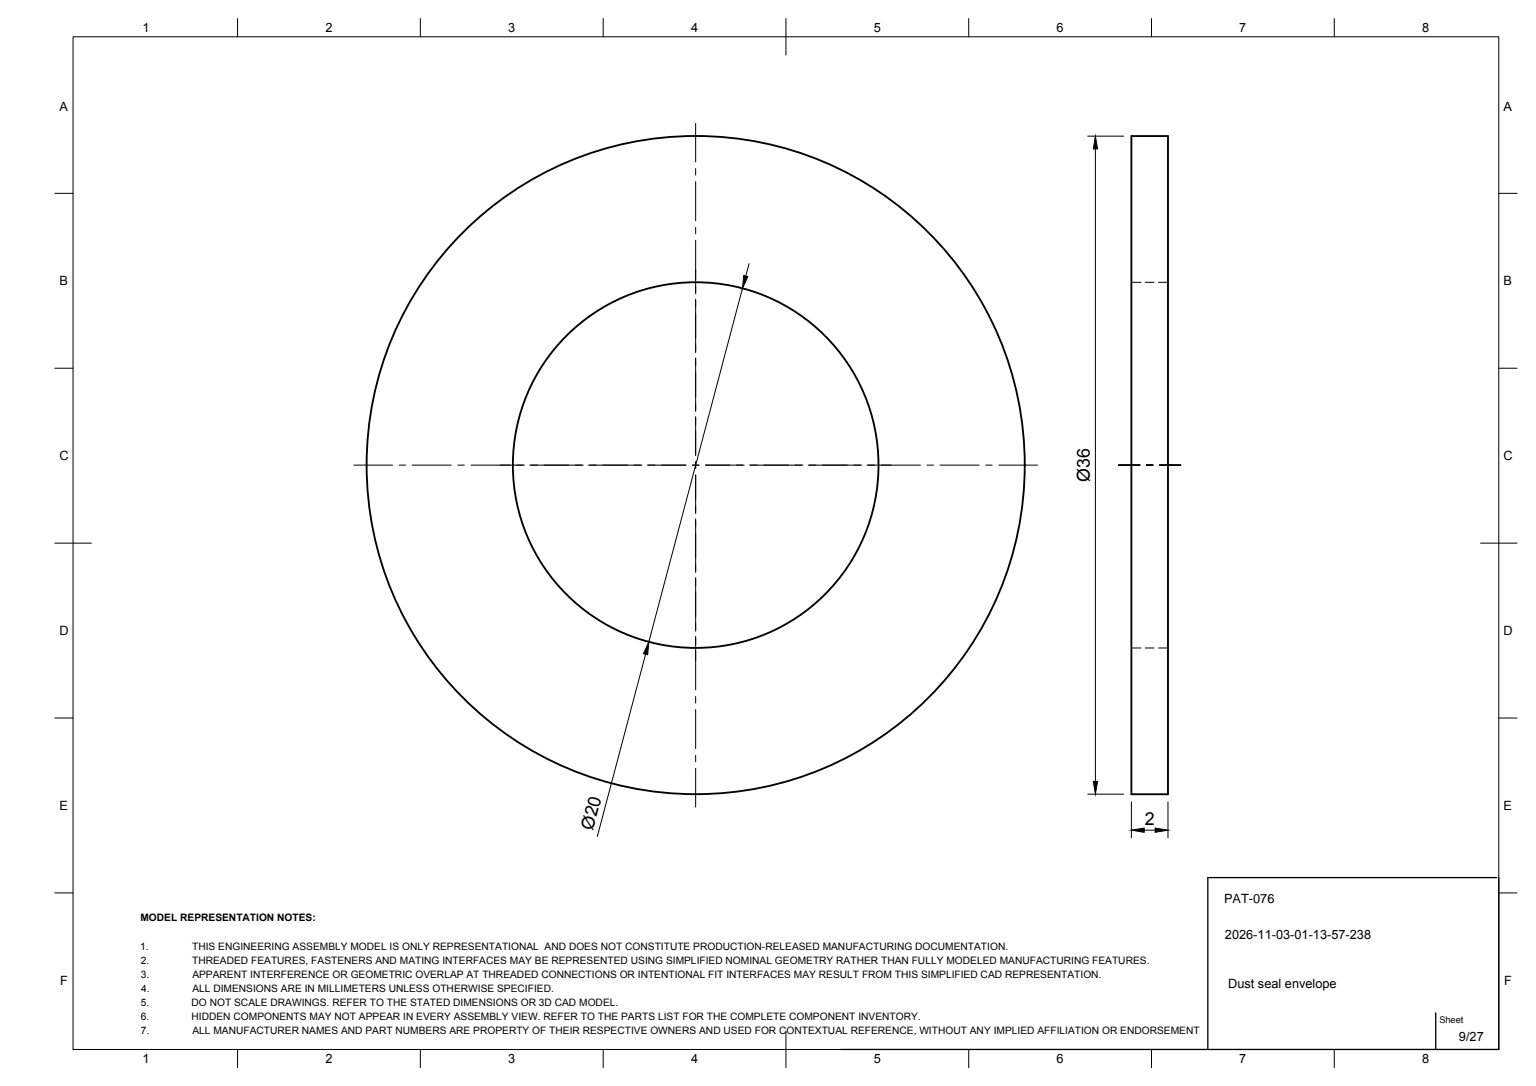
ISO-10303-21;
HEADER;
/* Generated by software containing ST-Developer
 * from STEP Tools, Inc. (www.steptools.com) 
 */

FILE_DESCRIPTION(
/* description */ ('Overhung pulley bearing cartridge'),
/* implementation_level */ '2;1');

FILE_NAME(
/* name */ 'Dust seal envelope.step',
/* time_stamp */ '2026-10-28T03:22:33-07:00',
/* author */ (''),
/* organization */ (''),
/* preprocessor_version */ 'ST-DEVELOPER v20.2',
/* originating_system */ 'Autodesk Translation Framework v15.17.0.0',
/* authorisation */ '');

FILE_SCHEMA (('AUTOMOTIVE_DESIGN { 1 0 10303 214 3 1 1 }'));
ENDSEC;

DATA;
#10=MECHANICAL_DESIGN_GEOMETRIC_PRESENTATION_REPRESENTATION('',(#287),#10963);
#243=SHAPE_REPRESENTATION_RELATIONSHIP('SRR','None',#11063,#265);
#265=ADVANCED_BREP_SHAPE_REPRESENTATION('',(#317),#10943);
#287=STYLED_ITEM('',(#11260),#317);
#317=MANIFOLD_SOLID_BREP('Body1',#5654);
#383=FACE_BOUND('',#1019,.T.);
#384=FACE_BOUND('',#1021,.T.);
#474=PLANE('',#6070);
#475=PLANE('',#6071);
#645=FACE_OUTER_BOUND('',#1016,.T.);
#646=FACE_OUTER_BOUND('',#1017,.T.);
#647=FACE_OUTER_BOUND('',#1018,.T.);
#648=FACE_OUTER_BOUND('',#1020,.T.);
#1016=EDGE_LOOP('',(#3933,#3934,#3935,#3936));
#1017=EDGE_LOOP('',(#3937,#3938,#3939,#3940));
#1018=EDGE_LOOP('',(#3941));
#1019=EDGE_LOOP('',(#3942));
#1020=EDGE_LOOP('',(#3943));
#1021=EDGE_LOOP('',(#3944));
#1404=LINE('',#8867,#1746);
#1405=LINE('',#8873,#1747);
#1746=VECTOR('',#7046,1.);
#1747=VECTOR('',#7053,1.8);
#2076=CIRCLE('',#6065,1.);
#2077=CIRCLE('',#6066,1.);
#2078=CIRCLE('',#6068,1.8);
#2079=CIRCLE('',#6069,1.8);
#2475=VERTEX_POINT('',#8864);
#2476=VERTEX_POINT('',#8866);
#2477=VERTEX_POINT('',#8870);
#2478=VERTEX_POINT('',#8872);
#3036=EDGE_CURVE('',#2475,#2475,#2076,.T.);
#3037=EDGE_CURVE('',#2475,#2476,#1404,.T.);
#3038=EDGE_CURVE('',#2476,#2476,#2077,.T.);
#3039=EDGE_CURVE('',#2477,#2477,#2078,.T.);
#3040=EDGE_CURVE('',#2477,#2478,#1405,.T.);
#3041=EDGE_CURVE('',#2478,#2478,#2079,.T.);
#3933=ORIENTED_EDGE('',*,*,#3036,.F.);
#3934=ORIENTED_EDGE('',*,*,#3037,.T.);
#3935=ORIENTED_EDGE('',*,*,#3038,.T.);
#3936=ORIENTED_EDGE('',*,*,#3037,.F.);
#3937=ORIENTED_EDGE('',*,*,#3039,.F.);
#3938=ORIENTED_EDGE('',*,*,#3040,.T.);
#3939=ORIENTED_EDGE('',*,*,#3041,.T.);
#3940=ORIENTED_EDGE('',*,*,#3040,.F.);
#3941=ORIENTED_EDGE('',*,*,#3039,.T.);
#3942=ORIENTED_EDGE('',*,*,#3036,.T.);
#3943=ORIENTED_EDGE('',*,*,#3041,.F.);
#3944=ORIENTED_EDGE('',*,*,#3038,.F.);
#5195=CYLINDRICAL_SURFACE('',#6064,1.);
#5196=CYLINDRICAL_SURFACE('',#6067,1.8);
#5389=ADVANCED_FACE('',(#645),#5195,.F.);
#5390=ADVANCED_FACE('',(#646),#5196,.T.);
#5391=ADVANCED_FACE('',(#647,#383),#474,.T.);
#5392=ADVANCED_FACE('',(#648,#384),#475,.F.);
#5654=CLOSED_SHELL('',(#5389,#5390,#5391,#5392));
#6063=AXIS2_PLACEMENT_3D('',#8862,#7040,#7041);
#6064=AXIS2_PLACEMENT_3D('',#8863,#7042,#7043);
#6065=AXIS2_PLACEMENT_3D('',#8865,#7044,#7045);
#6066=AXIS2_PLACEMENT_3D('',#8868,#7047,#7048);
#6067=AXIS2_PLACEMENT_3D('',#8869,#7049,#7050);
#6068=AXIS2_PLACEMENT_3D('',#8871,#7051,#7052);
#6069=AXIS2_PLACEMENT_3D('',#8874,#7054,#7055);
#6070=AXIS2_PLACEMENT_3D('',#8875,#7056,#7057);
#6071=AXIS2_PLACEMENT_3D('',#8876,#7058,#7059);
#7040=DIRECTION('axis',(0.,0.,1.));
#7041=DIRECTION('refdir',(1.,0.,0.));
#7042=DIRECTION('center_axis',(0.,1.,0.));
#7043=DIRECTION('ref_axis',(1.,0.,0.));
#7044=DIRECTION('center_axis',(0.,-1.,0.));
#7045=DIRECTION('ref_axis',(1.,0.,0.));
#7046=DIRECTION('',(0.,-1.,0.));
#7047=DIRECTION('center_axis',(0.,-1.,0.));
#7048=DIRECTION('ref_axis',(1.,0.,0.));
#7049=DIRECTION('center_axis',(0.,1.,0.));
#7050=DIRECTION('ref_axis',(1.,0.,0.));
#7051=DIRECTION('center_axis',(0.,1.,0.));
#7052=DIRECTION('ref_axis',(1.,0.,0.));
#7053=DIRECTION('',(0.,-1.,0.));
#7054=DIRECTION('center_axis',(0.,1.,0.));
#7055=DIRECTION('ref_axis',(1.,0.,0.));
#7056=DIRECTION('center_axis',(0.,1.,0.));
#7057=DIRECTION('ref_axis',(1.,0.,0.));
#7058=DIRECTION('center_axis',(0.,1.,0.));
#7059=DIRECTION('ref_axis',(1.,0.,0.));
#8862=CARTESIAN_POINT('',(0.,0.,0.));
#8863=CARTESIAN_POINT('Origin',(0.,-0.4,4.5));
#8864=CARTESIAN_POINT('',(-1.,-0.2,4.5));
#8865=CARTESIAN_POINT('Origin',(0.,-0.2,4.5));
#8866=CARTESIAN_POINT('',(-1.,-0.4,4.5));
#8867=CARTESIAN_POINT('',(-1.,-0.4,4.5));
#8868=CARTESIAN_POINT('Origin',(0.,-0.4,4.5));
#8869=CARTESIAN_POINT('Origin',(0.,-0.4,4.5));
#8870=CARTESIAN_POINT('',(-1.8,-0.2,4.5));
#8871=CARTESIAN_POINT('Origin',(0.,-0.2,4.5));
#8872=CARTESIAN_POINT('',(-1.8,-0.4,4.5));
#8873=CARTESIAN_POINT('',(-1.8,-0.4,4.5));
#8874=CARTESIAN_POINT('Origin',(0.,-0.4,4.5));
#8875=CARTESIAN_POINT('Origin',(0.,-0.2,4.5));
#8876=CARTESIAN_POINT('Origin',(0.,-0.4,4.5));
#10916=UNCERTAINTY_MEASURE_WITH_UNIT(LENGTH_MEASURE(0.001),#10964,
'DISTANCE_ACCURACY_VALUE',
'Maximum model space distance between geometric entities at asserted c
onnectivities');
#10936=UNCERTAINTY_MEASURE_WITH_UNIT(LENGTH_MEASURE(0.001),#10964,
'DISTANCE_ACCURACY_VALUE',
'Maximum model space distance between geometric entities at asserted c
onnectivities');
#10943=(
GEOMETRIC_REPRESENTATION_CONTEXT(3)
GLOBAL_UNCERTAINTY_ASSIGNED_CONTEXT((#10916))
GLOBAL_UNIT_ASSIGNED_CONTEXT((#10964,#10966,#10967))
REPRESENTATION_CONTEXT('','3D')
);
#10963=(
GEOMETRIC_REPRESENTATION_CONTEXT(3)
GLOBAL_UNCERTAINTY_ASSIGNED_CONTEXT((#10936))
GLOBAL_UNIT_ASSIGNED_CONTEXT((#10964,#10966,#10967))
REPRESENTATION_CONTEXT('','3D')
);
#10964=(
LENGTH_UNIT()
NAMED_UNIT(*)
SI_UNIT(.CENTI.,.METRE.)
);
#10966=(
NAMED_UNIT(*)
PLANE_ANGLE_UNIT()
SI_UNIT($,.RADIAN.)
);
#10967=(
NAMED_UNIT(*)
SI_UNIT($,.STERADIAN.)
SOLID_ANGLE_UNIT()
);
#10974=SHAPE_DEFINITION_REPRESENTATION(#11000,#11063);
#11000=PRODUCT_DEFINITION_SHAPE('',$,#11090);
#11063=SHAPE_REPRESENTATION('',(#6063),#10943);
#11083=PRODUCT_DEFINITION_CONTEXT('part definition',#11163,'design');
#11090=PRODUCT_DEFINITION('Dust seal envelope','Dust seal envelope',#11116,
#11083);
#11116=PRODUCT_DEFINITION_FORMATION('',$,#11171);
#11163=APPLICATION_CONTEXT(
'Core Data for Automotive Mechanical Design Process');
#11164=PRODUCT_CONTEXT('part definition',#11163,'mechanical');
#11171=PRODUCT('Dust seal envelope','Dust seal envelope',
'Dust seal envelope',(#11164));
#11254=COLOUR_RGB('Black',0.12,0.14,0.17);
#11255=FILL_AREA_STYLE_COLOUR('',#11254);
#11256=FILL_AREA_STYLE('',(#11255));
#11257=SURFACE_STYLE_FILL_AREA(#11256);
#11258=SURFACE_SIDE_STYLE('',(#11257));
#11259=SURFACE_STYLE_USAGE(.BOTH.,#11258);
#11260=PRESENTATION_STYLE_ASSIGNMENT((#11259));
ENDSEC;
END-ISO-10303-21;
